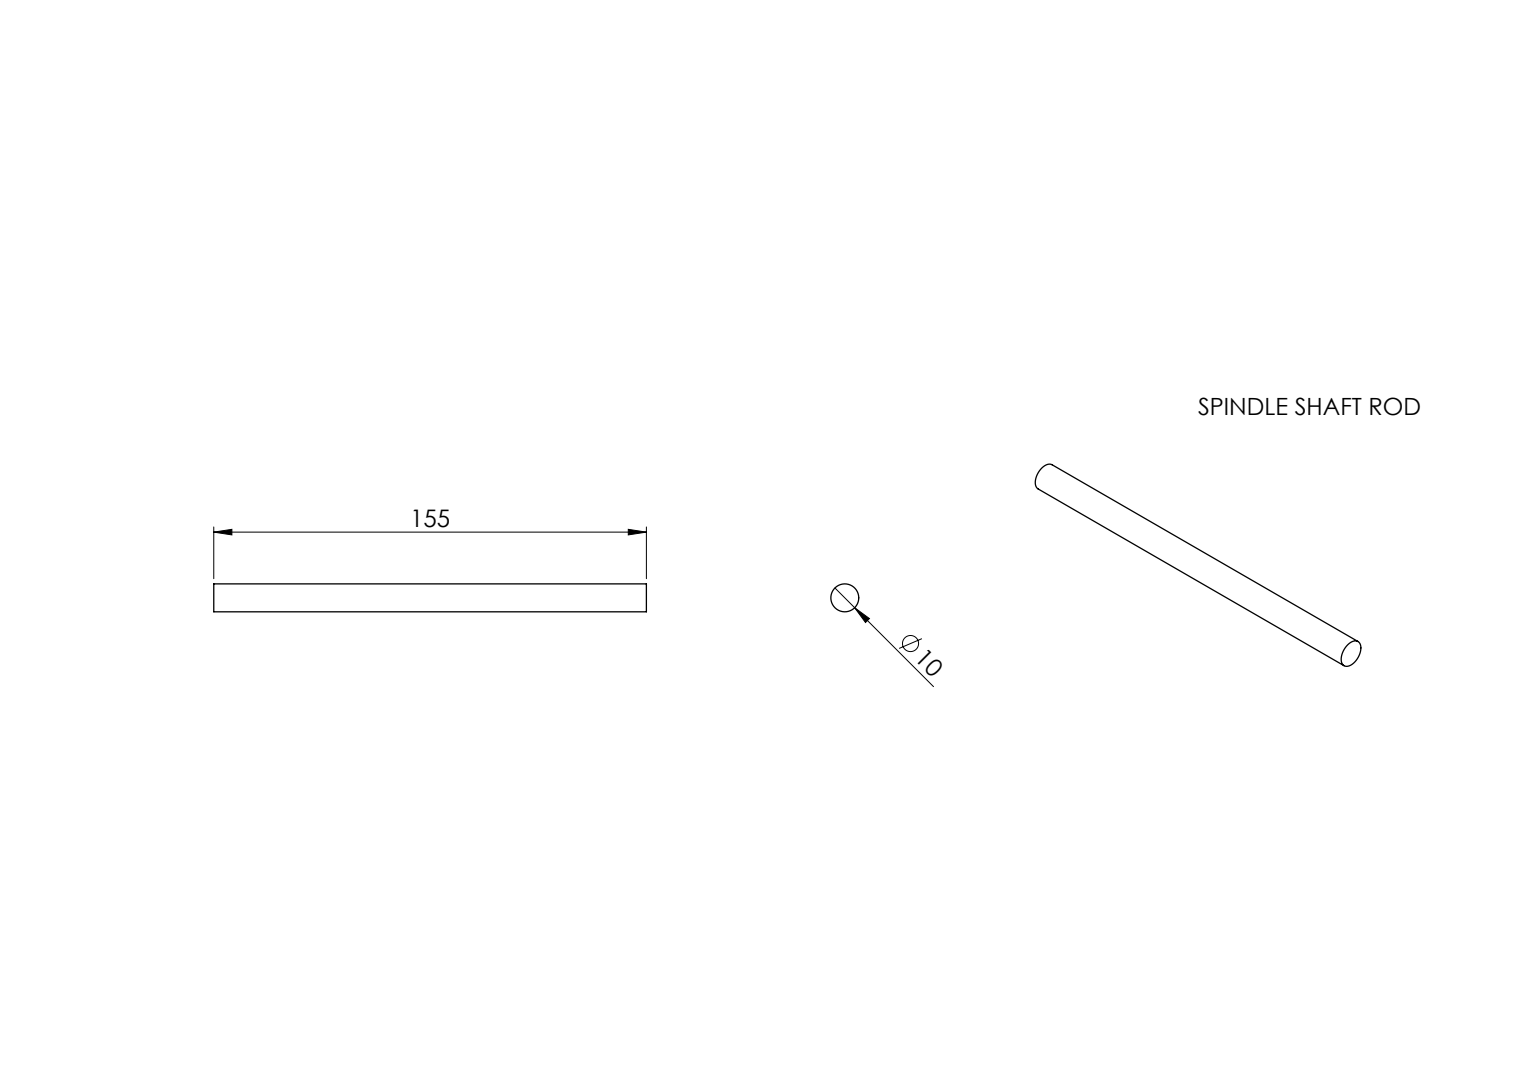
ISO-10303-21;
HEADER;
FILE_DESCRIPTION (('STEP AP214'),
    '1' );
FILE_NAME ('Spindle Shaft Rod.step',
    '2026-10-22T12:35:56',
    ( '' ),
    ( '' ),
    'SwSTEP 2.0',
    'SolidWorks 2026',
    '' );
FILE_SCHEMA (( 'AUTOMOTIVE_DESIGN' ));
ENDSEC;

DATA;
#19=PRODUCT_DEFINITION_FORMATION_WITH_SPECIFIED_SOURCE ( 'ANY', '', #2257, .NOT_KNOWN. ) ;
#62=ADVANCED_FACE ( 'NONE', ( #2597 ), #606, .F. ) ;
#67=CIRCLE ( 'NONE', #2220, 5.000000000000000000 ) ;
#98=DIRECTION ( 'NONE',  ( 0.000000000000000000, 0.000000000000000000, -1.000000000000000000 ) ) ;
#156=SURFACE_STYLE_USAGE ( .BOTH. , #409 ) ;
#243=APPLICATION_CONTEXT ( 'automotive_design' ) ;
#253=PRODUCT_CONTEXT ( 'NONE', #2801, 'mechanical' ) ;
#274=EDGE_CURVE ( 'NONE', #3069, #572, #2103, .T. ) ;
#330=SHAPE_REPRESENTATION ( 'Spindle Shaft Rod', ( #2878 ), #1321 ) ;
#345=DIRECTION ( 'NONE',  ( 1.000000000000000000, 0.000000000000000000, 0.000000000000000000 ) ) ;
#358=AXIS2_PLACEMENT_3D ( 'NONE', #894, #2425, #1157 ) ;
#376=ADVANCED_FACE ( 'NONE', ( #502 ), #991, .T. ) ;
#409=SURFACE_SIDE_STYLE ('',( #2405 ) ) ;
#425=( LENGTH_UNIT ( ) NAMED_UNIT ( * ) SI_UNIT ( .MILLI., .METRE. ) );
#465=EDGE_CURVE ( 'NONE', #572, #3069, #67, .T. ) ;
#472=CARTESIAN_POINT ( 'NONE',  ( -5.000000000000000000, -6.316519372592878167E-15, 12.50000000000000000 ) ) ;
#487=SHAPE_REPRESENTATION_RELATIONSHIP ( 'NONE' , 'NONE' ,  #330, #3045 ) ;
#502=FACE_OUTER_BOUND ( 'NONE', #3012, .T. ) ;
#539=ORIENTED_EDGE ( 'NONE', *, *, #274, .T. ) ;
#558=ORIENTED_EDGE ( 'NONE', *, *, #735, .T. ) ;
#572=VERTEX_POINT ( 'NONE', #1304 ) ;
#604=LINE ( 'NONE', #2391, #2518 ) ;
#606=PLANE ( 'NONE',  #1267 ) ;
#652=AXIS2_PLACEMENT_3D ( 'NONE', #1966, #1773, #964 ) ;
#700=DIRECTION ( 'NONE',  ( 1.000000000000000000, 0.000000000000000000, 0.000000000000000000 ) ) ;
#735=EDGE_CURVE ( 'NONE', #572, #1823, #604, .T. ) ;
#755=CARTESIAN_POINT ( 'NONE',  ( -5.000000000000000000, -6.928842772166554697E-15, 7.500000000000000000 ) ) ;
#771=ADVANCED_FACE ( 'NONE', ( #2358 ), #1893, .T. ) ;
#799=EDGE_CURVE ( 'NONE', #1823, #2935, #1473, .T. ) ;
#827=ADVANCED_FACE ( 'NONE', ( #1578 ), #3119, .T. ) ;
#894=CARTESIAN_POINT ( 'NONE',  ( 150.0000000000000000, -6.928842772166554697E-15, 7.500000000000000000 ) ) ;
#908=DIRECTION ( 'NONE',  ( 0.000000000000000000, 0.000000000000000000, -1.000000000000000000 ) ) ;
#921=EDGE_LOOP ( 'NONE', ( #2765, #975 ) ) ;
#925=( NAMED_UNIT ( * ) PLANE_ANGLE_UNIT ( ) SI_UNIT ( $, .RADIAN. ) );
#964=DIRECTION ( 'NONE',  ( 0.000000000000000000, 0.000000000000000000, -1.000000000000000000 ) ) ;
#975=ORIENTED_EDGE ( 'NONE', *, *, #274, .F. ) ;
#991=CYLINDRICAL_SURFACE ( 'NONE', #652, 5.000000000000000000 ) ;
#1024=CIRCLE ( 'NONE', #358, 5.000000000000000000 ) ;
#1025=ORIENTED_EDGE ( 'NONE', *, *, #465, .T. ) ;
#1026=EDGE_CURVE ( 'NONE', #3069, #2935, #1939, .T. ) ;
#1101=DIRECTION ( 'NONE',  ( 0.000000000000000000, 0.000000000000000000, -1.000000000000000000 ) ) ;
#1102=EDGE_LOOP ( 'NONE', ( #1025, #1417, #2065, #3212 ) ) ;
#1109=PRODUCT_DEFINITION_SHAPE ( 'NONE', 'NONE',  #3094 ) ;
#1115=COLOUR_RGB ( '',0.8941176470588234615, 0.8941176470588234615, 0.8941176470588234615 ) ;
#1138=FILL_AREA_STYLE_COLOUR ( '', #1115 ) ;
#1157=DIRECTION ( 'NONE',  ( 0.000000000000000000, 0.000000000000000000, -1.000000000000000000 ) ) ;
#1196=EDGE_LOOP ( 'NONE', ( #3078, #2672 ) ) ;
#1235=DIRECTION ( 'NONE',  ( 0.000000000000000000, 0.000000000000000000, -1.000000000000000000 ) ) ;
#1259=UNCERTAINTY_MEASURE_WITH_UNIT (LENGTH_MEASURE( 1.000000000000000082E-05 ), #2994, 'distance_accuracy_value', 'NONE');
#1267=AXIS2_PLACEMENT_3D ( 'NONE', #1382, #2155, #1101 ) ;
#1304=CARTESIAN_POINT ( 'NONE',  ( -5.000000000000000000, -6.928842772166554697E-15, 2.499999999999999556 ) ) ;
#1321=( GEOMETRIC_REPRESENTATION_CONTEXT ( 3 ) GLOBAL_UNCERTAINTY_ASSIGNED_CONTEXT ( ( #1687 ) ) GLOBAL_UNIT_ASSIGNED_CONTEXT ( ( #425, #1615, #1633 ) ) REPRESENTATION_CONTEXT ( 'NONE', 'WORKASPACE' ) );
#1371=ORIENTED_EDGE ( 'NONE', *, *, #1686, .F. ) ;
#1382=CARTESIAN_POINT ( 'NONE',  ( -5.000000000000000000, -6.928842772166554697E-15, 7.500000000000000000 ) ) ;
#1395=DIRECTION ( 'NONE',  ( 1.000000000000000000, 0.000000000000000000, 0.000000000000000000 ) ) ;
#1396=PRESENTATION_STYLE_ASSIGNMENT (( #156 ) ) ;
#1413=( LENGTH_UNIT ( ) NAMED_UNIT ( * ) SI_UNIT ( .MILLI., .METRE. ) );
#1417=ORIENTED_EDGE ( 'NONE', *, *, #1026, .T. ) ;
#1450=CARTESIAN_POINT ( 'NONE',  ( 150.0000000000000000, -6.928842772166554697E-15, 2.499999999999999556 ) ) ;
#1473=CIRCLE ( 'NONE', #2154, 5.000000000000000000 ) ;
#1484=DIRECTION ( 'NONE',  ( 1.000000000000000000, 0.000000000000000000, 0.000000000000000000 ) ) ;
#1515=( NAMED_UNIT ( * ) PLANE_ANGLE_UNIT ( ) SI_UNIT ( $, .RADIAN. ) );
#1578=FACE_OUTER_BOUND ( 'NONE', #1196, .T. ) ;
#1585=ORIENTED_EDGE ( 'NONE', *, *, #1026, .F. ) ;
#1615=( NAMED_UNIT ( * ) PLANE_ANGLE_UNIT ( ) SI_UNIT ( $, .RADIAN. ) );
#1633=( NAMED_UNIT ( * ) SI_UNIT ( $, .STERADIAN. ) SOLID_ANGLE_UNIT ( ) );
#1650=STYLED_ITEM ( 'NONE', ( #1396 ), #3045 ) ;
#1655=CARTESIAN_POINT ( 'NONE',  ( 150.0000000000000000, -6.928842772166554697E-15, 7.500000000000000000 ) ) ;
#1686=EDGE_CURVE ( 'NONE', #2935, #1823, #1024, .T. ) ;
#1687=UNCERTAINTY_MEASURE_WITH_UNIT (LENGTH_MEASURE( 1.000000000000000082E-05 ), #425, 'distance_accuracy_value', 'NONE');
#1727=DIRECTION ( 'NONE',  ( 1.000000000000000000, 0.000000000000000000, 0.000000000000000000 ) ) ;
#1773=DIRECTION ( 'NONE',  ( 1.000000000000000000, 0.000000000000000000, 0.000000000000000000 ) ) ;
#1809=PRODUCT_DEFINITION_CONTEXT ( 'detailed design', #243, 'design' ) ;
#1823=VERTEX_POINT ( 'NONE', #1450 ) ;
#1837=DIRECTION ( 'NONE',  ( 1.000000000000000000, 0.000000000000000000, 0.000000000000000000 ) ) ;
#1858=CARTESIAN_POINT ( 'NONE',  ( -5.000000000000000000, -6.928842772166554697E-15, 7.500000000000000000 ) ) ;
#1893=CYLINDRICAL_SURFACE ( 'NONE', #2979, 5.000000000000000000 ) ;
#1939=LINE ( 'NONE', #472, #1943 ) ;
#1943=VECTOR ( 'NONE', #700, 1000.000000000000000 ) ;
#1966=CARTESIAN_POINT ( 'NONE',  ( -5.000000000000000000, -6.928842772166554697E-15, 7.500000000000000000 ) ) ;
#2065=ORIENTED_EDGE ( 'NONE', *, *, #799, .F. ) ;
#2103=CIRCLE ( 'NONE', #2514, 5.000000000000000000 ) ;
#2137=DIRECTION ( 'NONE',  ( 1.000000000000000000, 0.000000000000000000, 0.000000000000000000 ) ) ;
#2154=AXIS2_PLACEMENT_3D ( 'NONE', #1655, #1395, #2611 ) ;
#2155=DIRECTION ( 'NONE',  ( 1.000000000000000000, 0.000000000000000000, 0.000000000000000000 ) ) ;
#2206=AXIS2_PLACEMENT_3D ( 'NONE', #3070, #345, #908 ) ;
#2210=MECHANICAL_DESIGN_GEOMETRIC_PRESENTATION_REPRESENTATION('',(#2723),#3038);
#2220=AXIS2_PLACEMENT_3D ( 'NONE', #755, #1727, #2243 ) ;
#2243=DIRECTION ( 'NONE',  ( 0.000000000000000000, 0.000000000000000000, -1.000000000000000000 ) ) ;
#2257=PRODUCT ( 'Spindle Shaft Rod', 'Spindle Shaft Rod', '', ( #253 ) ) ;
#2319=CARTESIAN_POINT ( 'NONE',  ( -5.000000000000000000, -6.316519372592878167E-15, 12.50000000000000000 ) ) ;
#2358=FACE_OUTER_BOUND ( 'NONE', #1102, .T. ) ;
#2391=CARTESIAN_POINT ( 'NONE',  ( -5.000000000000000000, -6.928842772166554697E-15, 2.499999999999999556 ) ) ;
#2405=SURFACE_STYLE_FILL_AREA ( #3122 ) ;
#2423=UNCERTAINTY_MEASURE_WITH_UNIT (LENGTH_MEASURE( 1.000000000000000082E-05 ), #1413, 'distance_accuracy_value', 'NONE');
#2425=DIRECTION ( 'NONE',  ( 1.000000000000000000, 0.000000000000000000, 0.000000000000000000 ) ) ;
#2457=CARTESIAN_POINT ( 'NONE',  ( -5.000000000000000000, -6.928842772166554697E-15, 7.500000000000000000 ) ) ;
#2514=AXIS2_PLACEMENT_3D ( 'NONE', #2457, #1484, #1235 ) ;
#2518=VECTOR ( 'NONE', #2826, 1000.000000000000000 ) ;
#2522=MECHANICAL_DESIGN_GEOMETRIC_PRESENTATION_REPRESENTATION('',(#1650),#2623);
#2548=( NAMED_UNIT ( * ) SI_UNIT ( $, .STERADIAN. ) SOLID_ANGLE_UNIT ( ) );
#2597=FACE_OUTER_BOUND ( 'NONE', #921, .T. ) ;
#2611=DIRECTION ( 'NONE',  ( 0.000000000000000000, 0.000000000000000000, -1.000000000000000000 ) ) ;
#2623=( GEOMETRIC_REPRESENTATION_CONTEXT ( 3 ) GLOBAL_UNCERTAINTY_ASSIGNED_CONTEXT ( ( #2423 ) ) GLOBAL_UNIT_ASSIGNED_CONTEXT ( ( #1413, #925, #2991 ) ) REPRESENTATION_CONTEXT ( 'NONE', 'WORKASPACE' ) );
#2661=SHAPE_DEFINITION_REPRESENTATION ( #1109, #330 ) ;
#2672=ORIENTED_EDGE ( 'NONE', *, *, #1686, .T. ) ;
#2723=STYLED_ITEM('',(#3257),#3192);
#2765=ORIENTED_EDGE ( 'NONE', *, *, #465, .F. ) ;
#2799=DIRECTION ( 'NONE',  ( 0.000000000000000000, 0.000000000000000000, 1.000000000000000000 ) ) ;
#2801=APPLICATION_CONTEXT ( 'automotive_design' ) ;
#2826=DIRECTION ( 'NONE',  ( 1.000000000000000000, 0.000000000000000000, 0.000000000000000000 ) ) ;
#2877=CLOSED_SHELL ( 'NONE', ( #771, #376, #62, #827 ) ) ;
#2878=AXIS2_PLACEMENT_3D ( 'NONE', #3071, #2799, #1837 ) ;
#2935=VERTEX_POINT ( 'NONE', #3110 ) ;
#2979=AXIS2_PLACEMENT_3D ( 'NONE', #1858, #2137, #98 ) ;
#2991=( NAMED_UNIT ( * ) SI_UNIT ( $, .STERADIAN. ) SOLID_ANGLE_UNIT ( ) );
#2994=( LENGTH_UNIT ( ) NAMED_UNIT ( * ) SI_UNIT ( .MILLI., .METRE. ) );
#3012=EDGE_LOOP ( 'NONE', ( #1585, #539, #558, #1371 ) ) ;
#3038=( GEOMETRIC_REPRESENTATION_CONTEXT ( 3 ) GLOBAL_UNCERTAINTY_ASSIGNED_CONTEXT ( ( #1259 ) ) GLOBAL_UNIT_ASSIGNED_CONTEXT ( ( #2994, #1515, #2548 ) ) REPRESENTATION_CONTEXT ( 'NONE', 'WORKASPACE' ) );
#3045=ADVANCED_BREP_SHAPE_REPRESENTATION ( '', ( #3192, #2878 ), #1321 ) ;
#3069=VERTEX_POINT ( 'NONE', #2319 ) ;
#3070=CARTESIAN_POINT ( 'NONE',  ( 150.0000000000000000, -6.928842772166554697E-15, 7.500000000000000000 ) ) ;
#3071=CARTESIAN_POINT ( 'NONE',  ( 0.000000000000000000, 0.000000000000000000, 0.000000000000000000 ) ) ;
#3078=ORIENTED_EDGE ( 'NONE', *, *, #799, .T. ) ;
#3094=PRODUCT_DEFINITION ( 'UNKNOWN', '', #19, #1809 ) ;
#3110=CARTESIAN_POINT ( 'NONE',  ( 150.0000000000000000, -6.316519372592878167E-15, 12.50000000000000000 ) ) ;
#3119=PLANE ( 'NONE',  #2206 ) ;
#3122=FILL_AREA_STYLE ('',( #1138 ) ) ;
#3192=MANIFOLD_SOLID_BREP ( 'Boss-Extrude1', #2877 ) ;
#3212=ORIENTED_EDGE ( 'NONE', *, *, #735, .F. ) ;
#3251=COLOUR_RGB('Grey',0.48,0.52,0.57);
#3252=FILL_AREA_STYLE_COLOUR('',#3251);
#3253=FILL_AREA_STYLE('',(#3252));
#3254=SURFACE_STYLE_FILL_AREA(#3253);
#3255=SURFACE_SIDE_STYLE('',(#3254));
#3256=SURFACE_STYLE_USAGE(.BOTH.,#3255);
#3257=PRESENTATION_STYLE_ASSIGNMENT((#3256));
ENDSEC;
END-ISO-10303-21;
